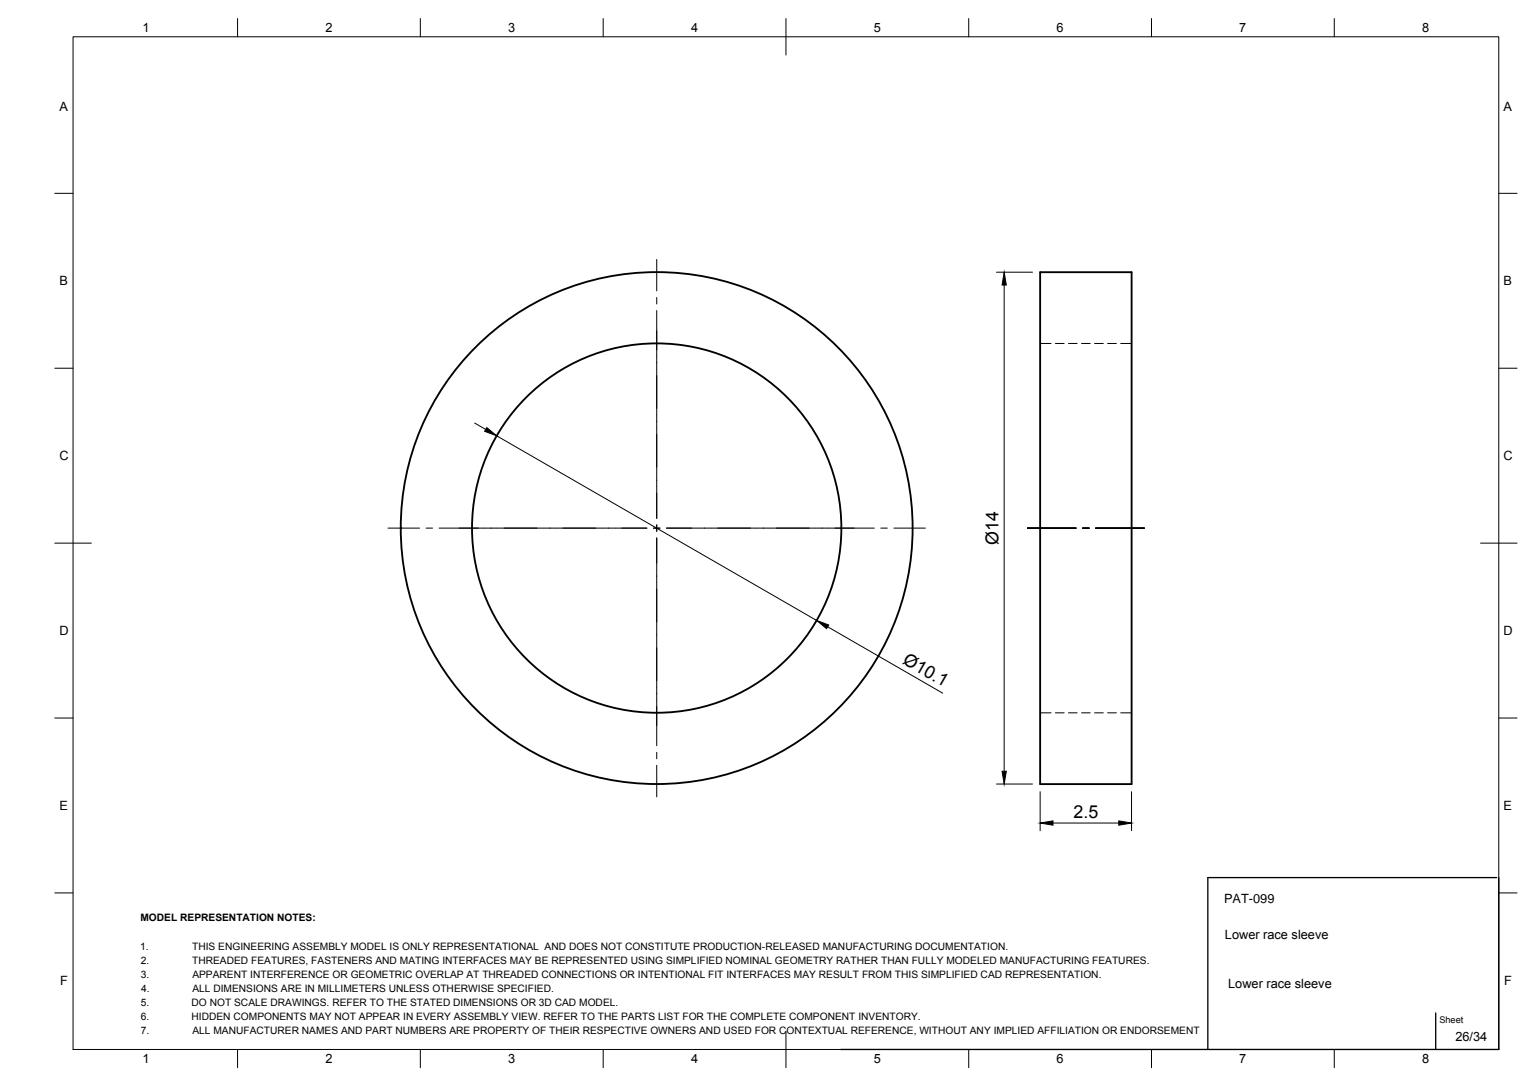
ISO-10303-21;
HEADER;
/* Generated by software containing ST-Developer
 * from STEP Tools, Inc. (www.steptools.com) 
 */

FILE_DESCRIPTION(
/* description */ ('PAT-099'),
/* implementation_level */ '2;1');

FILE_NAME(
/* name */ 'Lower race sleeve.step',
/* time_stamp */ '2026-10-29T17:25:42-07:00',
/* author */ (''),
/* organization */ (''),
/* preprocessor_version */ 'ST-DEVELOPER v20.2',
/* originating_system */ 'Autodesk Translation Framework v15.17.0.0',
/* authorisation */ '');

FILE_SCHEMA (('AUTOMOTIVE_DESIGN { 1 0 10303 214 3 1 1 }'));
ENDSEC;

DATA;
#10=MECHANICAL_DESIGN_GEOMETRIC_PRESENTATION_REPRESENTATION('',(#348),#11035);
#298=SHAPE_REPRESENTATION_RELATIONSHIP('SRR','None',#11168,#323);
#323=ADVANCED_BREP_SHAPE_REPRESENTATION('',(#380),#11018);
#348=STYLED_ITEM('',(#11372),#380);
#380=MANIFOLD_SOLID_BREP('Body1',#4717);
#493=FACE_BOUND('',#1190,.T.);
#494=FACE_BOUND('',#1192,.T.);
#595=PLANE('',#5361);
#596=PLANE('',#5362);
#814=FACE_OUTER_BOUND('',#1187,.T.);
#815=FACE_OUTER_BOUND('',#1188,.T.);
#816=FACE_OUTER_BOUND('',#1189,.T.);
#817=FACE_OUTER_BOUND('',#1191,.T.);
#1187=EDGE_LOOP('',(#3803,#3804,#3805,#3806));
#1188=EDGE_LOOP('',(#3807,#3808,#3809,#3810));
#1189=EDGE_LOOP('',(#3811));
#1190=EDGE_LOOP('',(#3812));
#1191=EDGE_LOOP('',(#3813));
#1192=EDGE_LOOP('',(#3814));
#1489=LINE('',#9956,#1741);
#1490=LINE('',#9962,#1742);
#1741=VECTOR('',#6496,0.505);
#1742=VECTOR('',#6503,0.7);
#2014=CIRCLE('',#5356,0.505);
#2015=CIRCLE('',#5357,0.505);
#2016=CIRCLE('',#5359,0.7);
#2017=CIRCLE('',#5360,0.7);
#2365=VERTEX_POINT('',#9953);
#2366=VERTEX_POINT('',#9955);
#2367=VERTEX_POINT('',#9959);
#2368=VERTEX_POINT('',#9961);
#2878=EDGE_CURVE('',#2365,#2365,#2014,.T.);
#2879=EDGE_CURVE('',#2365,#2366,#1489,.T.);
#2880=EDGE_CURVE('',#2366,#2366,#2015,.T.);
#2881=EDGE_CURVE('',#2367,#2367,#2016,.T.);
#2882=EDGE_CURVE('',#2367,#2368,#1490,.T.);
#2883=EDGE_CURVE('',#2368,#2368,#2017,.T.);
#3803=ORIENTED_EDGE('',*,*,#2878,.F.);
#3804=ORIENTED_EDGE('',*,*,#2879,.T.);
#3805=ORIENTED_EDGE('',*,*,#2880,.T.);
#3806=ORIENTED_EDGE('',*,*,#2879,.F.);
#3807=ORIENTED_EDGE('',*,*,#2881,.F.);
#3808=ORIENTED_EDGE('',*,*,#2882,.T.);
#3809=ORIENTED_EDGE('',*,*,#2883,.T.);
#3810=ORIENTED_EDGE('',*,*,#2882,.F.);
#3811=ORIENTED_EDGE('',*,*,#2881,.T.);
#3812=ORIENTED_EDGE('',*,*,#2878,.T.);
#3813=ORIENTED_EDGE('',*,*,#2883,.F.);
#3814=ORIENTED_EDGE('',*,*,#2880,.F.);
#4388=CYLINDRICAL_SURFACE('',#5355,0.505);
#4389=CYLINDRICAL_SURFACE('',#5358,0.7);
#4579=ADVANCED_FACE('',(#814),#4388,.F.);
#4580=ADVANCED_FACE('',(#815),#4389,.T.);
#4581=ADVANCED_FACE('',(#816,#493),#595,.T.);
#4582=ADVANCED_FACE('',(#817,#494),#596,.F.);
#4717=CLOSED_SHELL('',(#4579,#4580,#4581,#4582));
#5354=AXIS2_PLACEMENT_3D('',#9951,#6490,#6491);
#5355=AXIS2_PLACEMENT_3D('',#9952,#6492,#6493);
#5356=AXIS2_PLACEMENT_3D('',#9954,#6494,#6495);
#5357=AXIS2_PLACEMENT_3D('',#9957,#6497,#6498);
#5358=AXIS2_PLACEMENT_3D('',#9958,#6499,#6500);
#5359=AXIS2_PLACEMENT_3D('',#9960,#6501,#6502);
#5360=AXIS2_PLACEMENT_3D('',#9963,#6504,#6505);
#5361=AXIS2_PLACEMENT_3D('',#9964,#6506,#6507);
#5362=AXIS2_PLACEMENT_3D('',#9965,#6508,#6509);
#6490=DIRECTION('axis',(0.,0.,1.));
#6491=DIRECTION('refdir',(1.,0.,0.));
#6492=DIRECTION('center_axis',(0.,0.,1.));
#6493=DIRECTION('ref_axis',(1.,0.,0.));
#6494=DIRECTION('center_axis',(0.,0.,-1.));
#6495=DIRECTION('ref_axis',(1.,0.,0.));
#6496=DIRECTION('',(0.,0.,-1.));
#6497=DIRECTION('center_axis',(0.,0.,-1.));
#6498=DIRECTION('ref_axis',(1.,0.,0.));
#6499=DIRECTION('center_axis',(0.,0.,1.));
#6500=DIRECTION('ref_axis',(1.,0.,0.));
#6501=DIRECTION('center_axis',(0.,0.,1.));
#6502=DIRECTION('ref_axis',(1.,0.,0.));
#6503=DIRECTION('',(0.,0.,-1.));
#6504=DIRECTION('center_axis',(0.,0.,1.));
#6505=DIRECTION('ref_axis',(1.,0.,0.));
#6506=DIRECTION('center_axis',(0.,0.,1.));
#6507=DIRECTION('ref_axis',(1.,0.,0.));
#6508=DIRECTION('center_axis',(0.,0.,1.));
#6509=DIRECTION('ref_axis',(1.,0.,0.));
#9951=CARTESIAN_POINT('',(0.,0.,0.));
#9952=CARTESIAN_POINT('Origin',(0.,0.,1.8));
#9953=CARTESIAN_POINT('',(-0.505,-6.18446633569413E-17,2.05));
#9954=CARTESIAN_POINT('Origin',(0.,0.,2.05));
#9955=CARTESIAN_POINT('',(-0.505,-6.18446633569413E-17,1.8));
#9956=CARTESIAN_POINT('',(-0.505,-6.18446633569413E-17,1.8));
#9957=CARTESIAN_POINT('Origin',(0.,0.,1.8));
#9958=CARTESIAN_POINT('Origin',(0.,0.,1.8));
#9959=CARTESIAN_POINT('',(-0.7,-8.57252759403147E-17,2.05));
#9960=CARTESIAN_POINT('Origin',(0.,0.,2.05));
#9961=CARTESIAN_POINT('',(-0.7,-8.57252759403147E-17,1.8));
#9962=CARTESIAN_POINT('',(-0.7,-8.57252759403147E-17,1.8));
#9963=CARTESIAN_POINT('Origin',(0.,0.,1.8));
#9964=CARTESIAN_POINT('Origin',(0.,0.,2.05));
#9965=CARTESIAN_POINT('Origin',(0.,0.,1.8));
#10985=UNCERTAINTY_MEASURE_WITH_UNIT(LENGTH_MEASURE(0.001),#11036,
'DISTANCE_ACCURACY_VALUE',
'Maximum model space distance between geometric entities at asserted c
onnectivities');
#11002=UNCERTAINTY_MEASURE_WITH_UNIT(LENGTH_MEASURE(0.001),#11036,
'DISTANCE_ACCURACY_VALUE',
'Maximum model space distance between geometric entities at asserted c
onnectivities');
#11018=(
GEOMETRIC_REPRESENTATION_CONTEXT(3)
GLOBAL_UNCERTAINTY_ASSIGNED_CONTEXT((#10985))
GLOBAL_UNIT_ASSIGNED_CONTEXT((#11036,#11038,#11039))
REPRESENTATION_CONTEXT('','3D')
);
#11035=(
GEOMETRIC_REPRESENTATION_CONTEXT(3)
GLOBAL_UNCERTAINTY_ASSIGNED_CONTEXT((#11002))
GLOBAL_UNIT_ASSIGNED_CONTEXT((#11036,#11038,#11039))
REPRESENTATION_CONTEXT('','3D')
);
#11036=(
LENGTH_UNIT()
NAMED_UNIT(*)
SI_UNIT(.CENTI.,.METRE.)
);
#11038=(
NAMED_UNIT(*)
PLANE_ANGLE_UNIT()
SI_UNIT($,.RADIAN.)
);
#11039=(
NAMED_UNIT(*)
SI_UNIT($,.STERADIAN.)
SOLID_ANGLE_UNIT()
);
#11055=SHAPE_DEFINITION_REPRESENTATION(#11089,#11168);
#11089=PRODUCT_DEFINITION_SHAPE('',$,#11201);
#11168=SHAPE_REPRESENTATION('',(#5354),#11018);
#11185=PRODUCT_DEFINITION_CONTEXT('part definition',#11283,'design');
#11201=PRODUCT_DEFINITION('Lower race sleeve','Lower race sleeve',#11233,
#11185);
#11233=PRODUCT_DEFINITION_FORMATION('',$,#11300);
#11283=APPLICATION_CONTEXT(
'Core Data for Automotive Mechanical Design Process');
#11284=PRODUCT_CONTEXT('part definition',#11283,'mechanical');
#11300=PRODUCT('Lower race sleeve','Lower race sleeve',
'Lower race sleeve',(#11284));
#11366=COLOUR_RGB('Light Blue',0.38,0.62,0.78);
#11367=FILL_AREA_STYLE_COLOUR('',#11366);
#11368=FILL_AREA_STYLE('',(#11367));
#11369=SURFACE_STYLE_FILL_AREA(#11368);
#11370=SURFACE_SIDE_STYLE('',(#11369));
#11371=SURFACE_STYLE_USAGE(.BOTH.,#11370);
#11372=PRESENTATION_STYLE_ASSIGNMENT((#11371));
ENDSEC;
END-ISO-10303-21;
